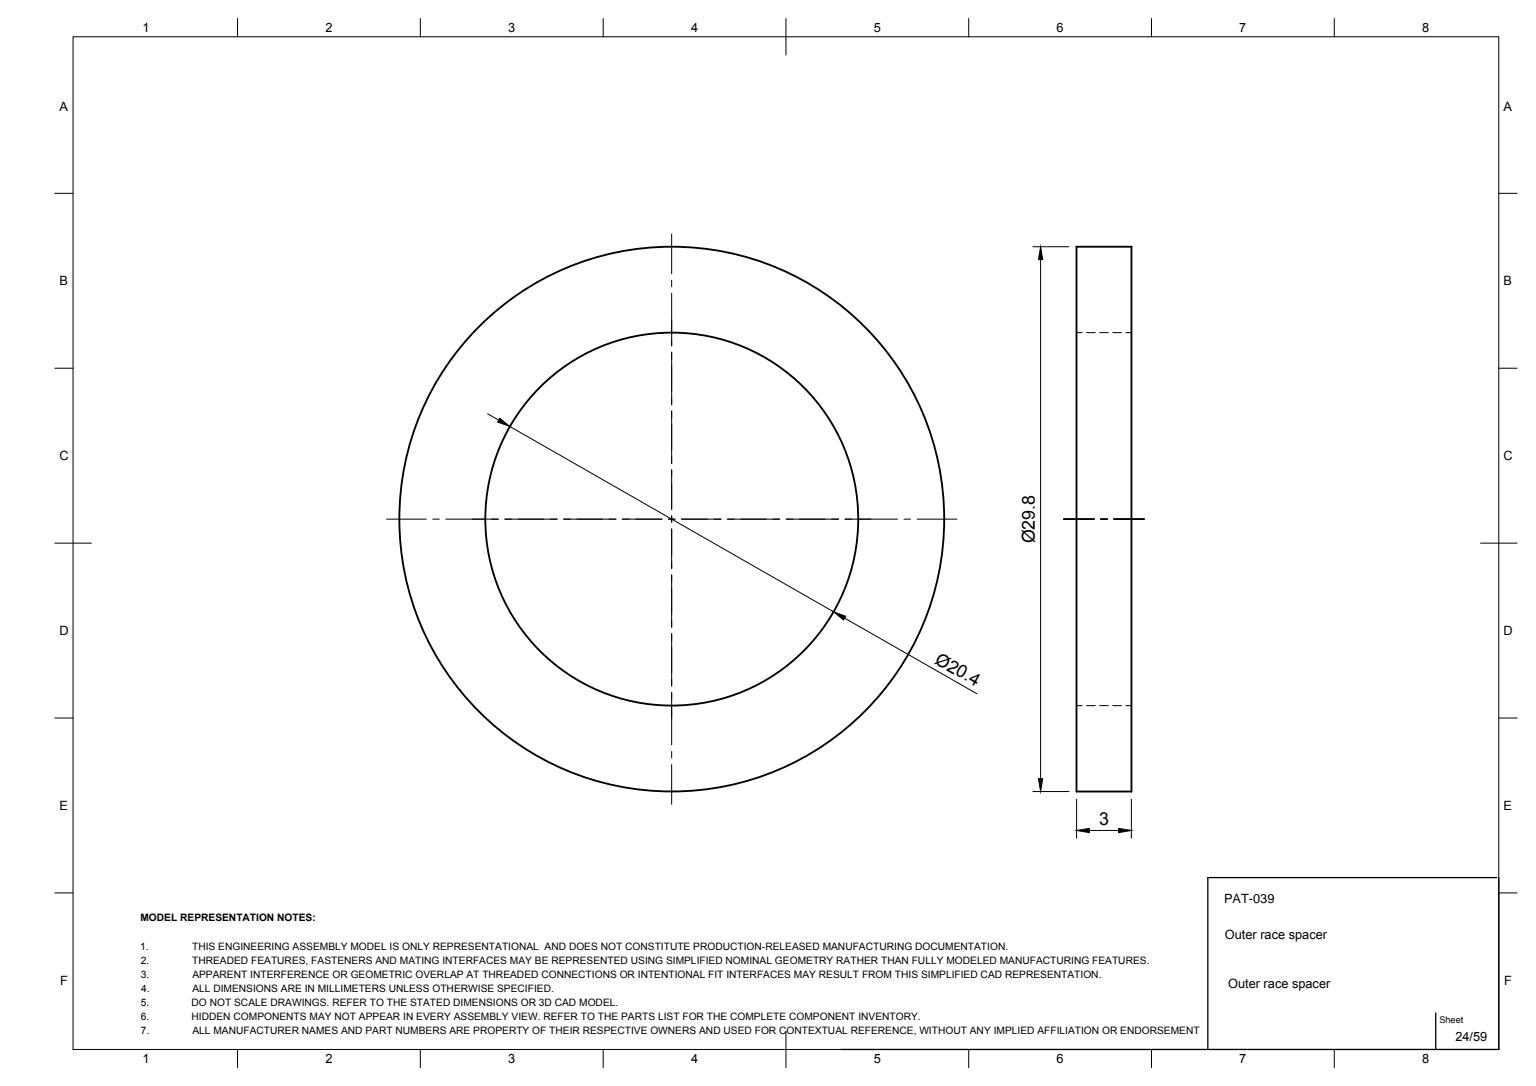
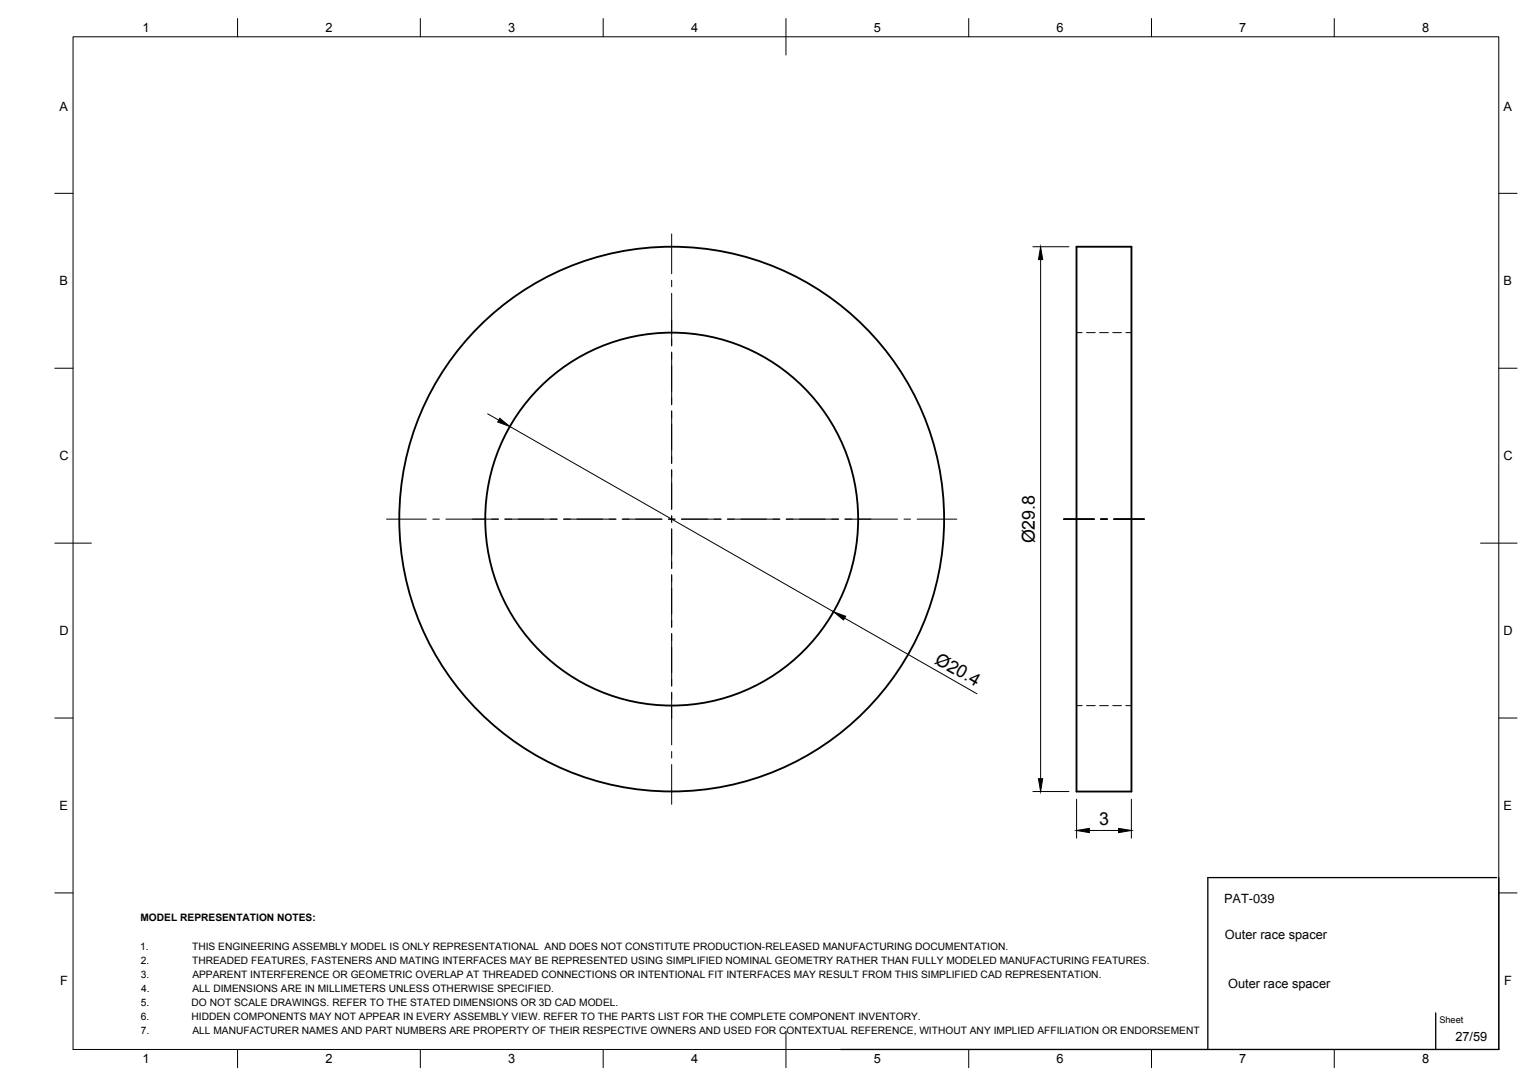
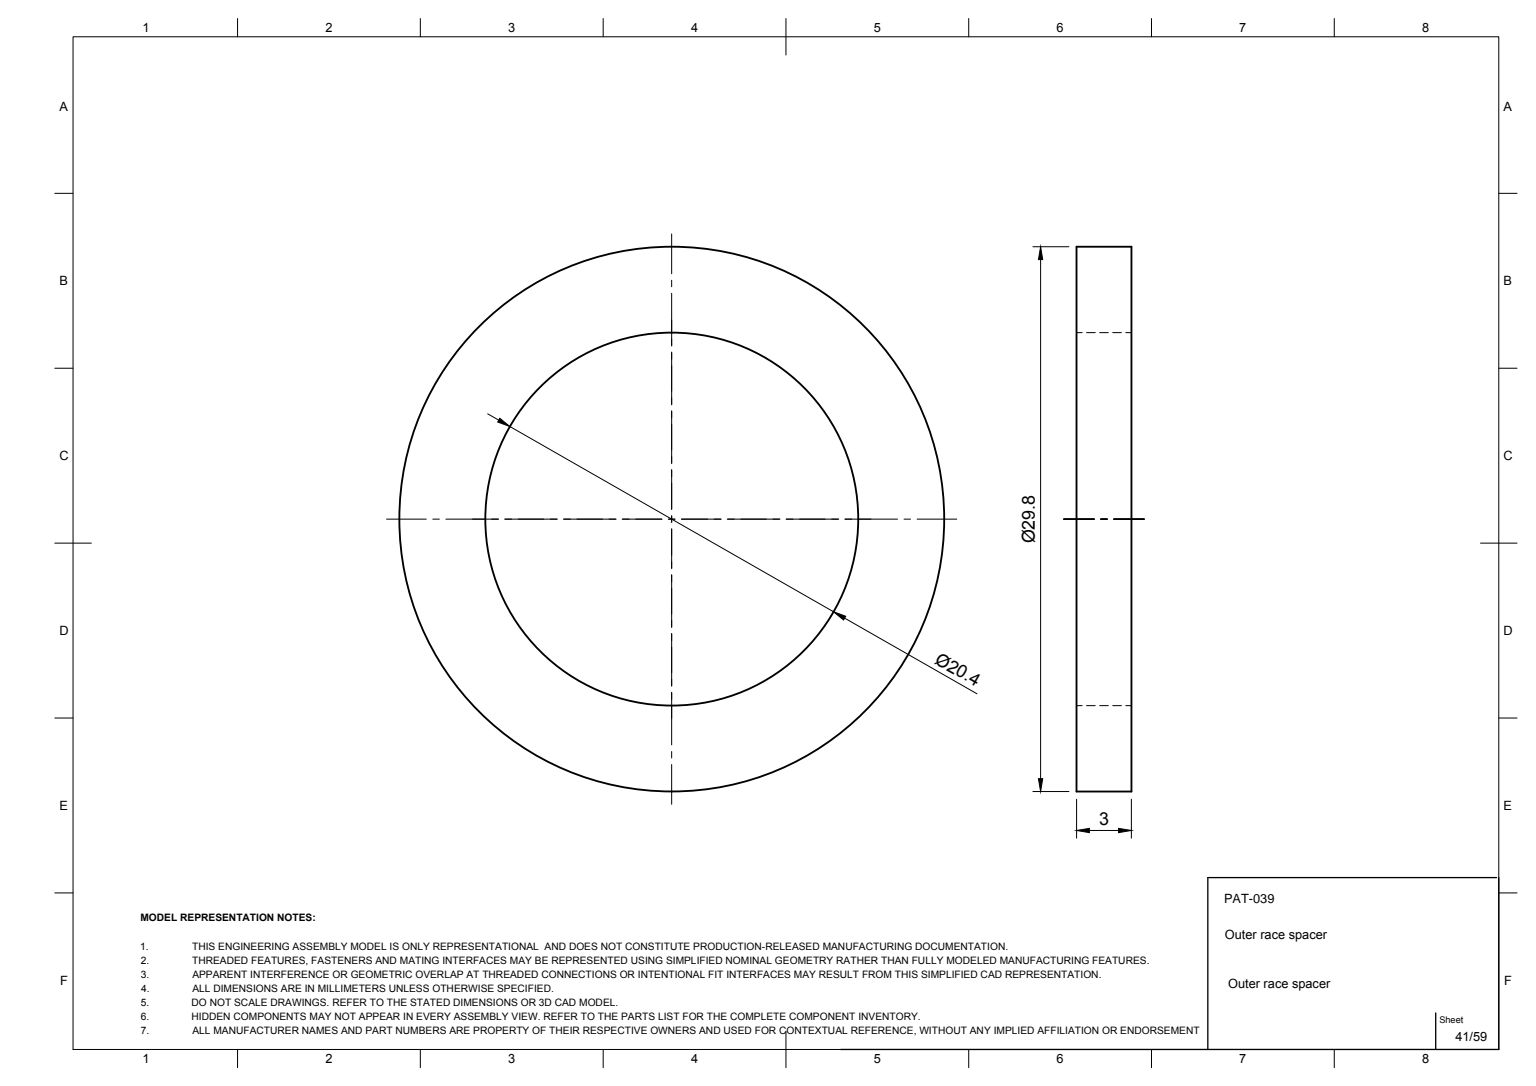
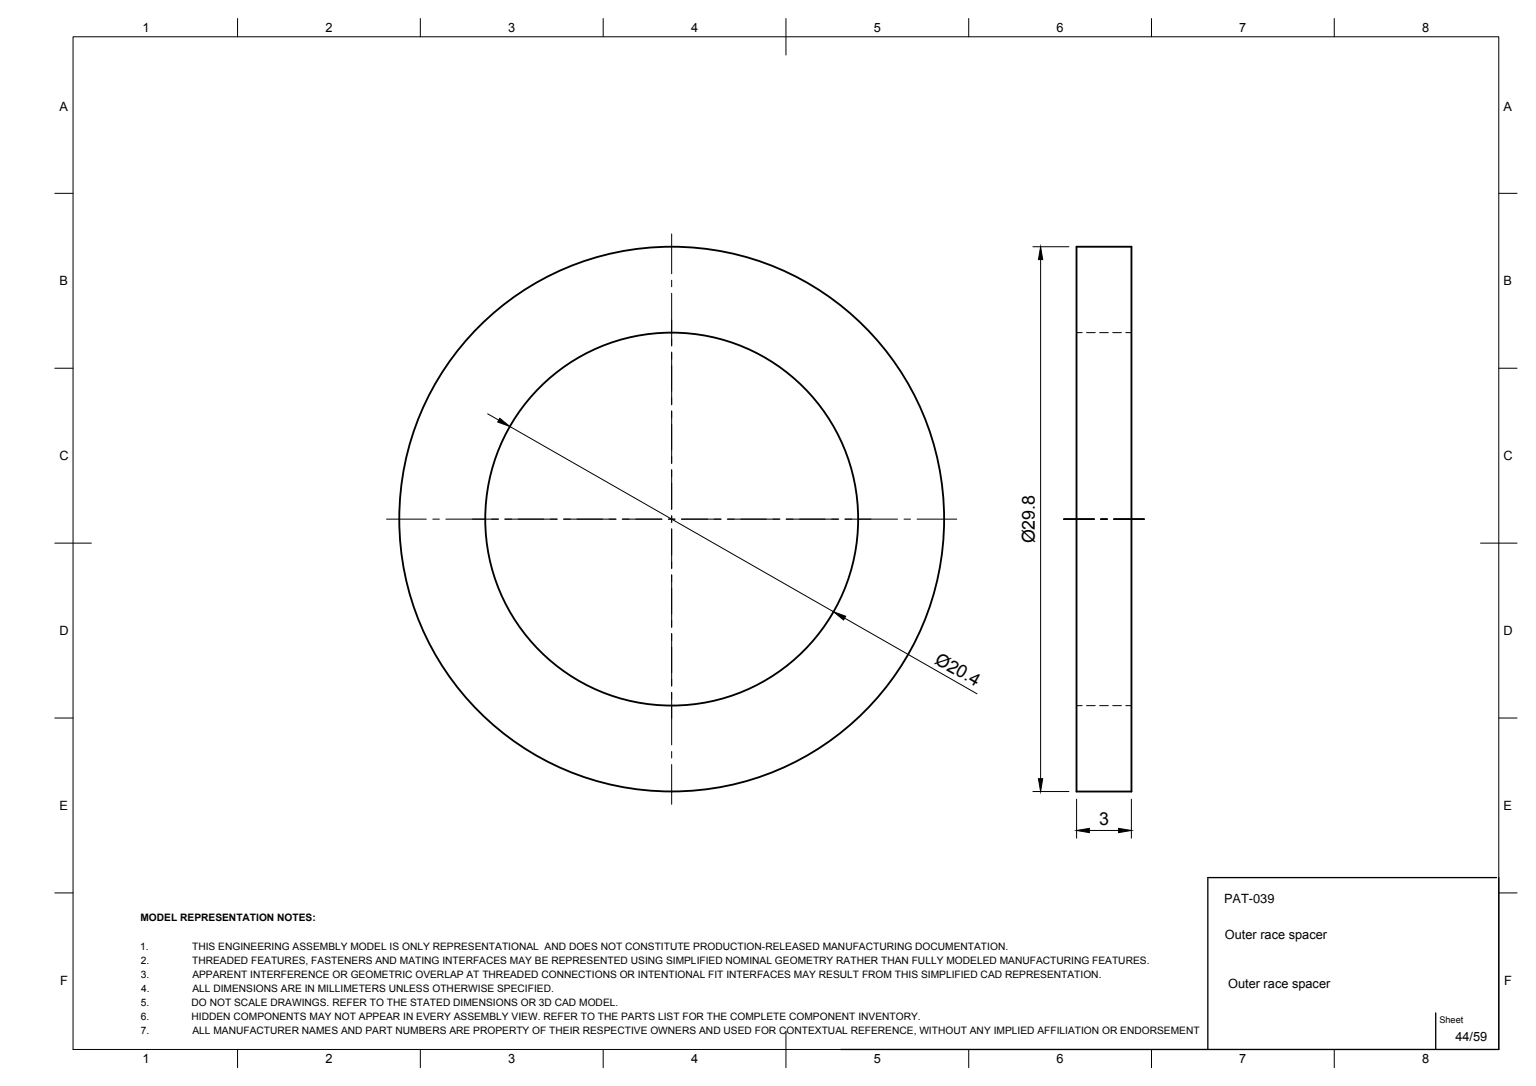
ISO-10303-21;
HEADER;
/* Generated by software containing ST-Developer
 * from STEP Tools, Inc. (www.steptools.com) 
 */

FILE_DESCRIPTION(
/* description */ ('Four-bar parallelogram arm'),
/* implementation_level */ '2;1');

FILE_NAME(
/* name */ 'Outer race spacer.step',
/* time_stamp */ '2026-10-28T03:24:55-07:00',
/* author */ (''),
/* organization */ (''),
/* preprocessor_version */ 'ST-DEVELOPER v20.2',
/* originating_system */ 'Autodesk Translation Framework v15.17.0.0',
/* authorisation */ '');

FILE_SCHEMA (('AUTOMOTIVE_DESIGN { 1 0 10303 214 3 1 1 }'));
ENDSEC;

DATA;
#10=MECHANICAL_DESIGN_GEOMETRIC_PRESENTATION_REPRESENTATION('',(#640),#14512);
#540=SHAPE_REPRESENTATION_RELATIONSHIP('SRR','None',#14762,#590);
#590=ADVANCED_BREP_SHAPE_REPRESENTATION('',(#697),#14477);
#640=STYLED_ITEM('',(#15087),#697);
#697=MANIFOLD_SOLID_BREP('Body1',#7345);
#827=FACE_BOUND('',#1872,.T.);
#828=FACE_BOUND('',#1874,.T.);
#1093=PLANE('',#8257);
#1094=PLANE('',#8258);
#1357=FACE_OUTER_BOUND('',#1869,.T.);
#1358=FACE_OUTER_BOUND('',#1870,.T.);
#1359=FACE_OUTER_BOUND('',#1871,.T.);
#1360=FACE_OUTER_BOUND('',#1873,.T.);
#1869=EDGE_LOOP('',(#5634,#5635,#5636,#5637));
#1870=EDGE_LOOP('',(#5638,#5639,#5640,#5641));
#1871=EDGE_LOOP('',(#5642));
#1872=EDGE_LOOP('',(#5643));
#1873=EDGE_LOOP('',(#5644));
#1874=EDGE_LOOP('',(#5645));
#2493=LINE('',#12748,#2887);
#2494=LINE('',#12754,#2888);
#2887=VECTOR('',#9781,1.02);
#2888=VECTOR('',#9788,1.49);
#3236=CIRCLE('',#8252,1.02);
#3237=CIRCLE('',#8253,1.02);
#3238=CIRCLE('',#8255,1.49);
#3239=CIRCLE('',#8256,1.49);
#3758=VERTEX_POINT('',#12745);
#3759=VERTEX_POINT('',#12747);
#3760=VERTEX_POINT('',#12751);
#3761=VERTEX_POINT('',#12753);
#4448=EDGE_CURVE('',#3758,#3758,#3236,.T.);
#4449=EDGE_CURVE('',#3758,#3759,#2493,.T.);
#4450=EDGE_CURVE('',#3759,#3759,#3237,.T.);
#4451=EDGE_CURVE('',#3760,#3760,#3238,.T.);
#4452=EDGE_CURVE('',#3760,#3761,#2494,.T.);
#4453=EDGE_CURVE('',#3761,#3761,#3239,.T.);
#5634=ORIENTED_EDGE('',*,*,#4448,.F.);
#5635=ORIENTED_EDGE('',*,*,#4449,.T.);
#5636=ORIENTED_EDGE('',*,*,#4450,.T.);
#5637=ORIENTED_EDGE('',*,*,#4449,.F.);
#5638=ORIENTED_EDGE('',*,*,#4451,.F.);
#5639=ORIENTED_EDGE('',*,*,#4452,.T.);
#5640=ORIENTED_EDGE('',*,*,#4453,.T.);
#5641=ORIENTED_EDGE('',*,*,#4452,.F.);
#5642=ORIENTED_EDGE('',*,*,#4451,.T.);
#5643=ORIENTED_EDGE('',*,*,#4448,.T.);
#5644=ORIENTED_EDGE('',*,*,#4453,.F.);
#5645=ORIENTED_EDGE('',*,*,#4450,.F.);
#6779=CYLINDRICAL_SURFACE('',#8251,1.02);
#6780=CYLINDRICAL_SURFACE('',#8254,1.49);
#7062=ADVANCED_FACE('',(#1357),#6779,.F.);
#7063=ADVANCED_FACE('',(#1358),#6780,.T.);
#7064=ADVANCED_FACE('',(#1359,#827),#1093,.T.);
#7065=ADVANCED_FACE('',(#1360,#828),#1094,.F.);
#7345=CLOSED_SHELL('',(#7062,#7063,#7064,#7065));
#8250=AXIS2_PLACEMENT_3D('',#12743,#9775,#9776);
#8251=AXIS2_PLACEMENT_3D('',#12744,#9777,#9778);
#8252=AXIS2_PLACEMENT_3D('',#12746,#9779,#9780);
#8253=AXIS2_PLACEMENT_3D('',#12749,#9782,#9783);
#8254=AXIS2_PLACEMENT_3D('',#12750,#9784,#9785);
#8255=AXIS2_PLACEMENT_3D('',#12752,#9786,#9787);
#8256=AXIS2_PLACEMENT_3D('',#12755,#9789,#9790);
#8257=AXIS2_PLACEMENT_3D('',#12756,#9791,#9792);
#8258=AXIS2_PLACEMENT_3D('',#12757,#9793,#9794);
#9775=DIRECTION('axis',(0.,0.,1.));
#9776=DIRECTION('refdir',(1.,0.,0.));
#9777=DIRECTION('center_axis',(0.,1.,0.));
#9778=DIRECTION('ref_axis',(1.,0.,0.));
#9779=DIRECTION('center_axis',(0.,-1.,0.));
#9780=DIRECTION('ref_axis',(1.,0.,0.));
#9781=DIRECTION('',(0.,-1.,0.));
#9782=DIRECTION('center_axis',(0.,-1.,0.));
#9783=DIRECTION('ref_axis',(1.,0.,0.));
#9784=DIRECTION('center_axis',(0.,1.,0.));
#9785=DIRECTION('ref_axis',(1.,0.,0.));
#9786=DIRECTION('center_axis',(0.,1.,0.));
#9787=DIRECTION('ref_axis',(1.,0.,0.));
#9788=DIRECTION('',(0.,-1.,0.));
#9789=DIRECTION('center_axis',(0.,1.,0.));
#9790=DIRECTION('ref_axis',(1.,0.,0.));
#9791=DIRECTION('center_axis',(0.,1.,0.));
#9792=DIRECTION('ref_axis',(1.,0.,0.));
#9793=DIRECTION('center_axis',(0.,1.,0.));
#9794=DIRECTION('ref_axis',(1.,0.,0.));
#12743=CARTESIAN_POINT('',(0.,0.,0.));
#12744=CARTESIAN_POINT('Origin',(0.,-0.15,8.));
#12745=CARTESIAN_POINT('',(-1.02,0.15,8.));
#12746=CARTESIAN_POINT('Origin',(0.,0.15,8.));
#12747=CARTESIAN_POINT('',(-1.02,-0.15,8.));
#12748=CARTESIAN_POINT('',(-1.02,-0.15,8.));
#12749=CARTESIAN_POINT('Origin',(0.,-0.15,8.));
#12750=CARTESIAN_POINT('Origin',(0.,-0.15,8.));
#12751=CARTESIAN_POINT('',(-1.49,0.15,8.));
#12752=CARTESIAN_POINT('Origin',(0.,0.15,8.));
#12753=CARTESIAN_POINT('',(-1.49,-0.15,8.));
#12754=CARTESIAN_POINT('',(-1.49,-0.15,8.));
#12755=CARTESIAN_POINT('Origin',(0.,-0.15,8.));
#12756=CARTESIAN_POINT('Origin',(0.,0.15,8.));
#12757=CARTESIAN_POINT('Origin',(0.,-0.15,8.));
#14420=UNCERTAINTY_MEASURE_WITH_UNIT(LENGTH_MEASURE(0.001),#14513,
'DISTANCE_ACCURACY_VALUE',
'Maximum model space distance between geometric entities at asserted c
onnectivities');
#14455=UNCERTAINTY_MEASURE_WITH_UNIT(LENGTH_MEASURE(0.001),#14513,
'DISTANCE_ACCURACY_VALUE',
'Maximum model space distance between geometric entities at asserted c
onnectivities');
#14477=(
GEOMETRIC_REPRESENTATION_CONTEXT(3)
GLOBAL_UNCERTAINTY_ASSIGNED_CONTEXT((#14420))
GLOBAL_UNIT_ASSIGNED_CONTEXT((#14513,#14515,#14516))
REPRESENTATION_CONTEXT('','3D')
);
#14512=(
GEOMETRIC_REPRESENTATION_CONTEXT(3)
GLOBAL_UNCERTAINTY_ASSIGNED_CONTEXT((#14455))
GLOBAL_UNIT_ASSIGNED_CONTEXT((#14513,#14515,#14516))
REPRESENTATION_CONTEXT('','3D')
);
#14513=(
LENGTH_UNIT()
NAMED_UNIT(*)
SI_UNIT(.CENTI.,.METRE.)
);
#14515=(
NAMED_UNIT(*)
PLANE_ANGLE_UNIT()
SI_UNIT($,.RADIAN.)
);
#14516=(
NAMED_UNIT(*)
SI_UNIT($,.STERADIAN.)
SOLID_ANGLE_UNIT()
);
#14538=SHAPE_DEFINITION_REPRESENTATION(#14594,#14762);
#14594=PRODUCT_DEFINITION_SHAPE('',$,#14819);
#14762=SHAPE_REPRESENTATION('',(#8250),#14477);
#14797=PRODUCT_DEFINITION_CONTEXT('part definition',#14967,'design');
#14819=PRODUCT_DEFINITION('Outer race spacer','Outer race spacer',#14875,
#14797);
#14875=PRODUCT_DEFINITION_FORMATION('',$,#14990);
#14967=APPLICATION_CONTEXT(
'Core Data for Automotive Mechanical Design Process');
#14968=PRODUCT_CONTEXT('part definition',#14967,'mechanical');
#14990=PRODUCT('Outer race spacer','Outer race spacer',
'Outer race spacer',(#14968));
#15081=COLOUR_RGB('Grey',0.48,0.52,0.57);
#15082=FILL_AREA_STYLE_COLOUR('',#15081);
#15083=FILL_AREA_STYLE('',(#15082));
#15084=SURFACE_STYLE_FILL_AREA(#15083);
#15085=SURFACE_SIDE_STYLE('',(#15084));
#15086=SURFACE_STYLE_USAGE(.BOTH.,#15085);
#15087=PRESENTATION_STYLE_ASSIGNMENT((#15086));
ENDSEC;
END-ISO-10303-21;
